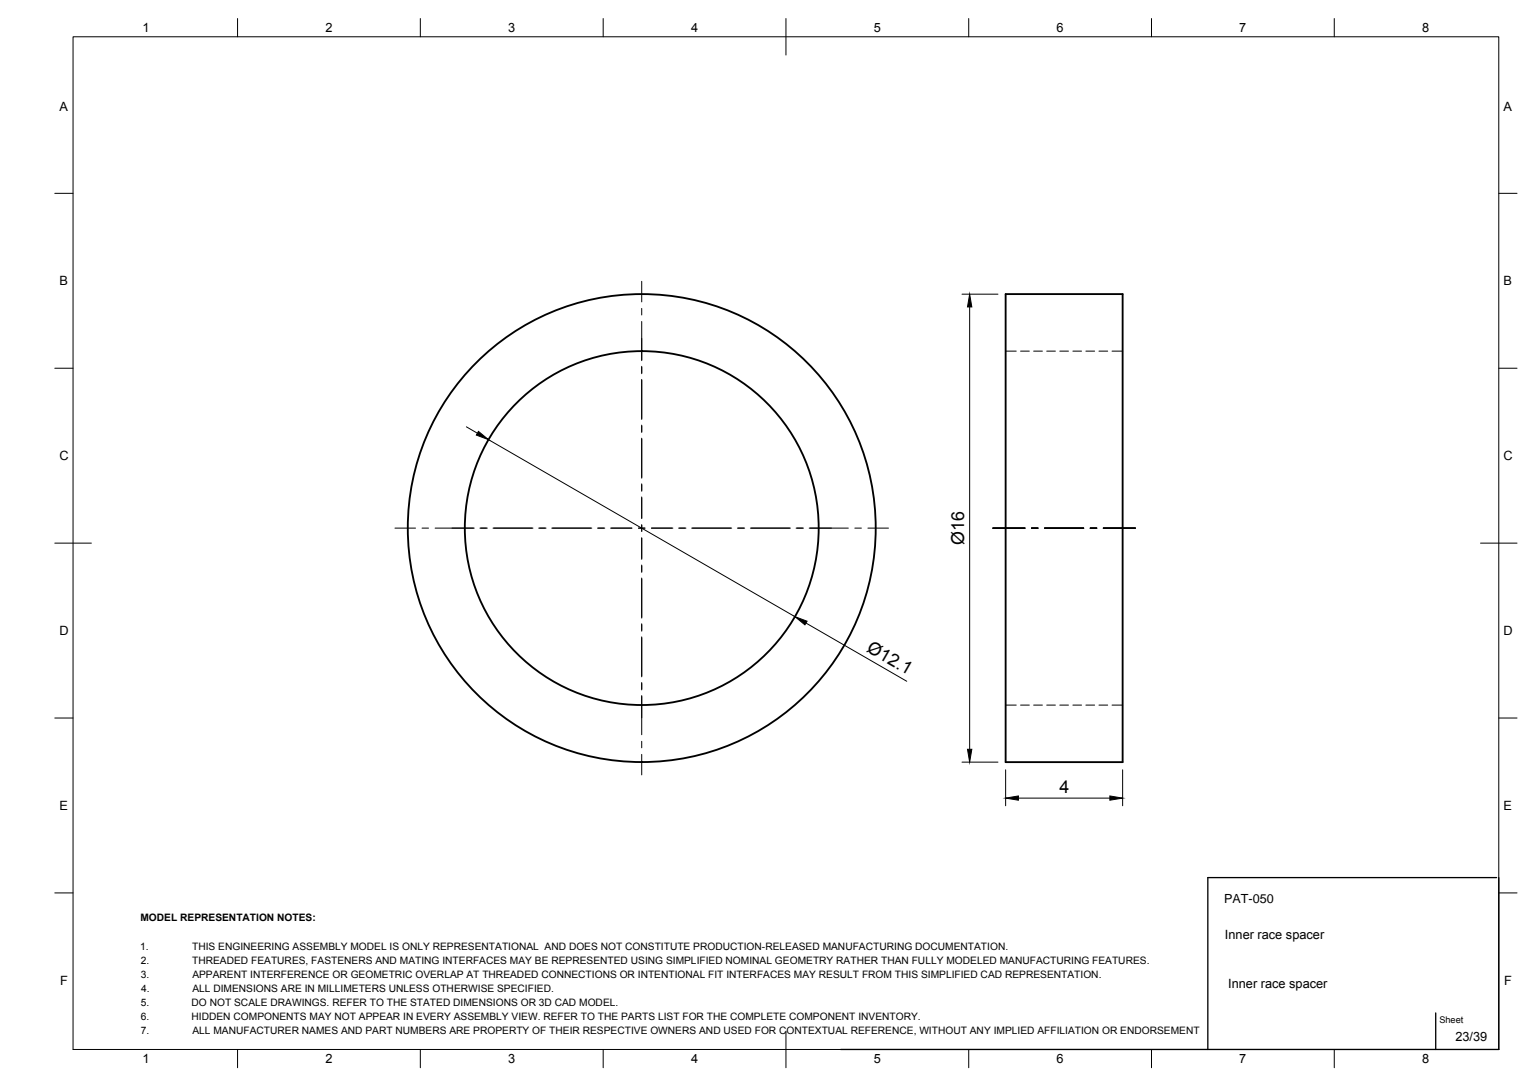
ISO-10303-21;
HEADER;
/* Generated by software containing ST-Developer
 * from STEP Tools, Inc. (www.steptools.com) 
 */

FILE_DESCRIPTION(
/* description */ ('Hand wheel with handle and shaft collar'),
/* implementation_level */ '2;1');

FILE_NAME(
/* name */ 'Inner race spacer.step',
/* time_stamp */ '2026-10-28T03:23:19-07:00',
/* author */ (''),
/* organization */ (''),
/* preprocessor_version */ 'ST-DEVELOPER v20.2',
/* originating_system */ 'Autodesk Translation Framework v15.17.0.0',
/* authorisation */ '');

FILE_SCHEMA (('AUTOMOTIVE_DESIGN { 1 0 10303 214 3 1 1 }'));
ENDSEC;

DATA;
#10=MECHANICAL_DESIGN_GEOMETRIC_PRESENTATION_REPRESENTATION('',(#418),#10510);
#347=SHAPE_REPRESENTATION_RELATIONSHIP('SRR','None',#10665,#379);
#379=ADVANCED_BREP_SHAPE_REPRESENTATION('',(#464),#10492);
#418=STYLED_ITEM('',(#10908),#464);
#464=MANIFOLD_SOLID_BREP('Body1',#5318);
#564=FACE_BOUND('',#1332,.T.);
#565=FACE_BOUND('',#1334,.T.);
#687=PLANE('',#6069);
#688=PLANE('',#6070);
#932=FACE_OUTER_BOUND('',#1329,.T.);
#933=FACE_OUTER_BOUND('',#1330,.T.);
#934=FACE_OUTER_BOUND('',#1331,.T.);
#935=FACE_OUTER_BOUND('',#1333,.T.);
#1329=EDGE_LOOP('',(#4303,#4304,#4305,#4306));
#1330=EDGE_LOOP('',(#4307,#4308,#4309,#4310));
#1331=EDGE_LOOP('',(#4311));
#1332=EDGE_LOOP('',(#4312));
#1333=EDGE_LOOP('',(#4313));
#1334=EDGE_LOOP('',(#4314));
#1697=LINE('',#9347,#2007);
#1698=LINE('',#9353,#2008);
#2007=VECTOR('',#7339,0.605);
#2008=VECTOR('',#7346,0.8);
#2304=CIRCLE('',#6064,0.605);
#2305=CIRCLE('',#6065,0.605);
#2306=CIRCLE('',#6067,0.8);
#2307=CIRCLE('',#6068,0.8);
#2700=VERTEX_POINT('',#9344);
#2701=VERTEX_POINT('',#9346);
#2702=VERTEX_POINT('',#9350);
#2703=VERTEX_POINT('',#9352);
#3269=EDGE_CURVE('',#2700,#2700,#2304,.T.);
#3270=EDGE_CURVE('',#2700,#2701,#1697,.T.);
#3271=EDGE_CURVE('',#2701,#2701,#2305,.T.);
#3272=EDGE_CURVE('',#2702,#2702,#2306,.T.);
#3273=EDGE_CURVE('',#2702,#2703,#1698,.T.);
#3274=EDGE_CURVE('',#2703,#2703,#2307,.T.);
#4303=ORIENTED_EDGE('',*,*,#3269,.F.);
#4304=ORIENTED_EDGE('',*,*,#3270,.T.);
#4305=ORIENTED_EDGE('',*,*,#3271,.T.);
#4306=ORIENTED_EDGE('',*,*,#3270,.F.);
#4307=ORIENTED_EDGE('',*,*,#3272,.F.);
#4308=ORIENTED_EDGE('',*,*,#3273,.T.);
#4309=ORIENTED_EDGE('',*,*,#3274,.T.);
#4310=ORIENTED_EDGE('',*,*,#3273,.F.);
#4311=ORIENTED_EDGE('',*,*,#3272,.T.);
#4312=ORIENTED_EDGE('',*,*,#3269,.T.);
#4313=ORIENTED_EDGE('',*,*,#3274,.F.);
#4314=ORIENTED_EDGE('',*,*,#3271,.F.);
#4936=CYLINDRICAL_SURFACE('',#6063,0.605);
#4937=CYLINDRICAL_SURFACE('',#6066,0.8);
#5144=ADVANCED_FACE('',(#932),#4936,.F.);
#5145=ADVANCED_FACE('',(#933),#4937,.T.);
#5146=ADVANCED_FACE('',(#934,#564),#687,.T.);
#5147=ADVANCED_FACE('',(#935,#565),#688,.F.);
#5318=CLOSED_SHELL('',(#5144,#5145,#5146,#5147));
#6062=AXIS2_PLACEMENT_3D('',#9342,#7333,#7334);
#6063=AXIS2_PLACEMENT_3D('',#9343,#7335,#7336);
#6064=AXIS2_PLACEMENT_3D('',#9345,#7337,#7338);
#6065=AXIS2_PLACEMENT_3D('',#9348,#7340,#7341);
#6066=AXIS2_PLACEMENT_3D('',#9349,#7342,#7343);
#6067=AXIS2_PLACEMENT_3D('',#9351,#7344,#7345);
#6068=AXIS2_PLACEMENT_3D('',#9354,#7347,#7348);
#6069=AXIS2_PLACEMENT_3D('',#9355,#7349,#7350);
#6070=AXIS2_PLACEMENT_3D('',#9356,#7351,#7352);
#7333=DIRECTION('axis',(0.,0.,1.));
#7334=DIRECTION('refdir',(1.,0.,0.));
#7335=DIRECTION('center_axis',(0.,1.,0.));
#7336=DIRECTION('ref_axis',(1.,0.,0.));
#7337=DIRECTION('center_axis',(0.,-1.,0.));
#7338=DIRECTION('ref_axis',(1.,0.,0.));
#7339=DIRECTION('',(0.,-1.,0.));
#7340=DIRECTION('center_axis',(0.,-1.,0.));
#7341=DIRECTION('ref_axis',(1.,0.,0.));
#7342=DIRECTION('center_axis',(0.,1.,0.));
#7343=DIRECTION('ref_axis',(1.,0.,0.));
#7344=DIRECTION('center_axis',(0.,1.,0.));
#7345=DIRECTION('ref_axis',(1.,0.,0.));
#7346=DIRECTION('',(0.,-1.,0.));
#7347=DIRECTION('center_axis',(0.,1.,0.));
#7348=DIRECTION('ref_axis',(1.,0.,0.));
#7349=DIRECTION('center_axis',(0.,1.,0.));
#7350=DIRECTION('ref_axis',(1.,0.,0.));
#7351=DIRECTION('center_axis',(0.,1.,0.));
#7352=DIRECTION('ref_axis',(1.,0.,0.));
#9342=CARTESIAN_POINT('',(0.,0.,0.));
#9343=CARTESIAN_POINT('Origin',(0.,4.5,10.));
#9344=CARTESIAN_POINT('',(-0.605,4.9,10.));
#9345=CARTESIAN_POINT('Origin',(0.,4.9,10.));
#9346=CARTESIAN_POINT('',(-0.605,4.5,10.));
#9347=CARTESIAN_POINT('',(-0.605,4.5,10.));
#9348=CARTESIAN_POINT('Origin',(0.,4.5,10.));
#9349=CARTESIAN_POINT('Origin',(0.,4.5,10.));
#9350=CARTESIAN_POINT('',(-0.8,4.9,10.));
#9351=CARTESIAN_POINT('Origin',(0.,4.9,10.));
#9352=CARTESIAN_POINT('',(-0.8,4.5,10.));
#9353=CARTESIAN_POINT('',(-0.8,4.5,10.));
#9354=CARTESIAN_POINT('Origin',(0.,4.5,10.));
#9355=CARTESIAN_POINT('Origin',(0.,4.9,10.));
#9356=CARTESIAN_POINT('Origin',(0.,4.5,10.));
#10453=UNCERTAINTY_MEASURE_WITH_UNIT(LENGTH_MEASURE(0.001),#10511,
'DISTANCE_ACCURACY_VALUE',
'Maximum model space distance between geometric entities at asserted c
onnectivities');
#10471=UNCERTAINTY_MEASURE_WITH_UNIT(LENGTH_MEASURE(0.001),#10511,
'DISTANCE_ACCURACY_VALUE',
'Maximum model space distance between geometric entities at asserted c
onnectivities');
#10492=(
GEOMETRIC_REPRESENTATION_CONTEXT(3)
GLOBAL_UNCERTAINTY_ASSIGNED_CONTEXT((#10453))
GLOBAL_UNIT_ASSIGNED_CONTEXT((#10511,#10513,#10514))
REPRESENTATION_CONTEXT('','3D')
);
#10510=(
GEOMETRIC_REPRESENTATION_CONTEXT(3)
GLOBAL_UNCERTAINTY_ASSIGNED_CONTEXT((#10471))
GLOBAL_UNIT_ASSIGNED_CONTEXT((#10511,#10513,#10514))
REPRESENTATION_CONTEXT('','3D')
);
#10511=(
LENGTH_UNIT()
NAMED_UNIT(*)
SI_UNIT(.CENTI.,.METRE.)
);
#10513=(
NAMED_UNIT(*)
PLANE_ANGLE_UNIT()
SI_UNIT($,.RADIAN.)
);
#10514=(
NAMED_UNIT(*)
SI_UNIT($,.STERADIAN.)
SOLID_ANGLE_UNIT()
);
#10535=SHAPE_DEFINITION_REPRESENTATION(#10578,#10665);
#10578=PRODUCT_DEFINITION_SHAPE('',$,#10704);
#10665=SHAPE_REPRESENTATION('',(#6062),#10492);
#10683=PRODUCT_DEFINITION_CONTEXT('part definition',#10799,'design');
#10704=PRODUCT_DEFINITION('Inner race spacer','Inner race spacer',#10742,
#10683);
#10742=PRODUCT_DEFINITION_FORMATION('',$,#10821);
#10799=APPLICATION_CONTEXT(
'Core Data for Automotive Mechanical Design Process');
#10800=PRODUCT_CONTEXT('part definition',#10799,'mechanical');
#10821=PRODUCT('Inner race spacer','Inner race spacer',
'Inner race spacer',(#10800));
#10902=COLOUR_RGB('Grey',0.48,0.52,0.57);
#10903=FILL_AREA_STYLE_COLOUR('',#10902);
#10904=FILL_AREA_STYLE('',(#10903));
#10905=SURFACE_STYLE_FILL_AREA(#10904);
#10906=SURFACE_SIDE_STYLE('',(#10905));
#10907=SURFACE_STYLE_USAGE(.BOTH.,#10906);
#10908=PRESENTATION_STYLE_ASSIGNMENT((#10907));
ENDSEC;
END-ISO-10303-21;
